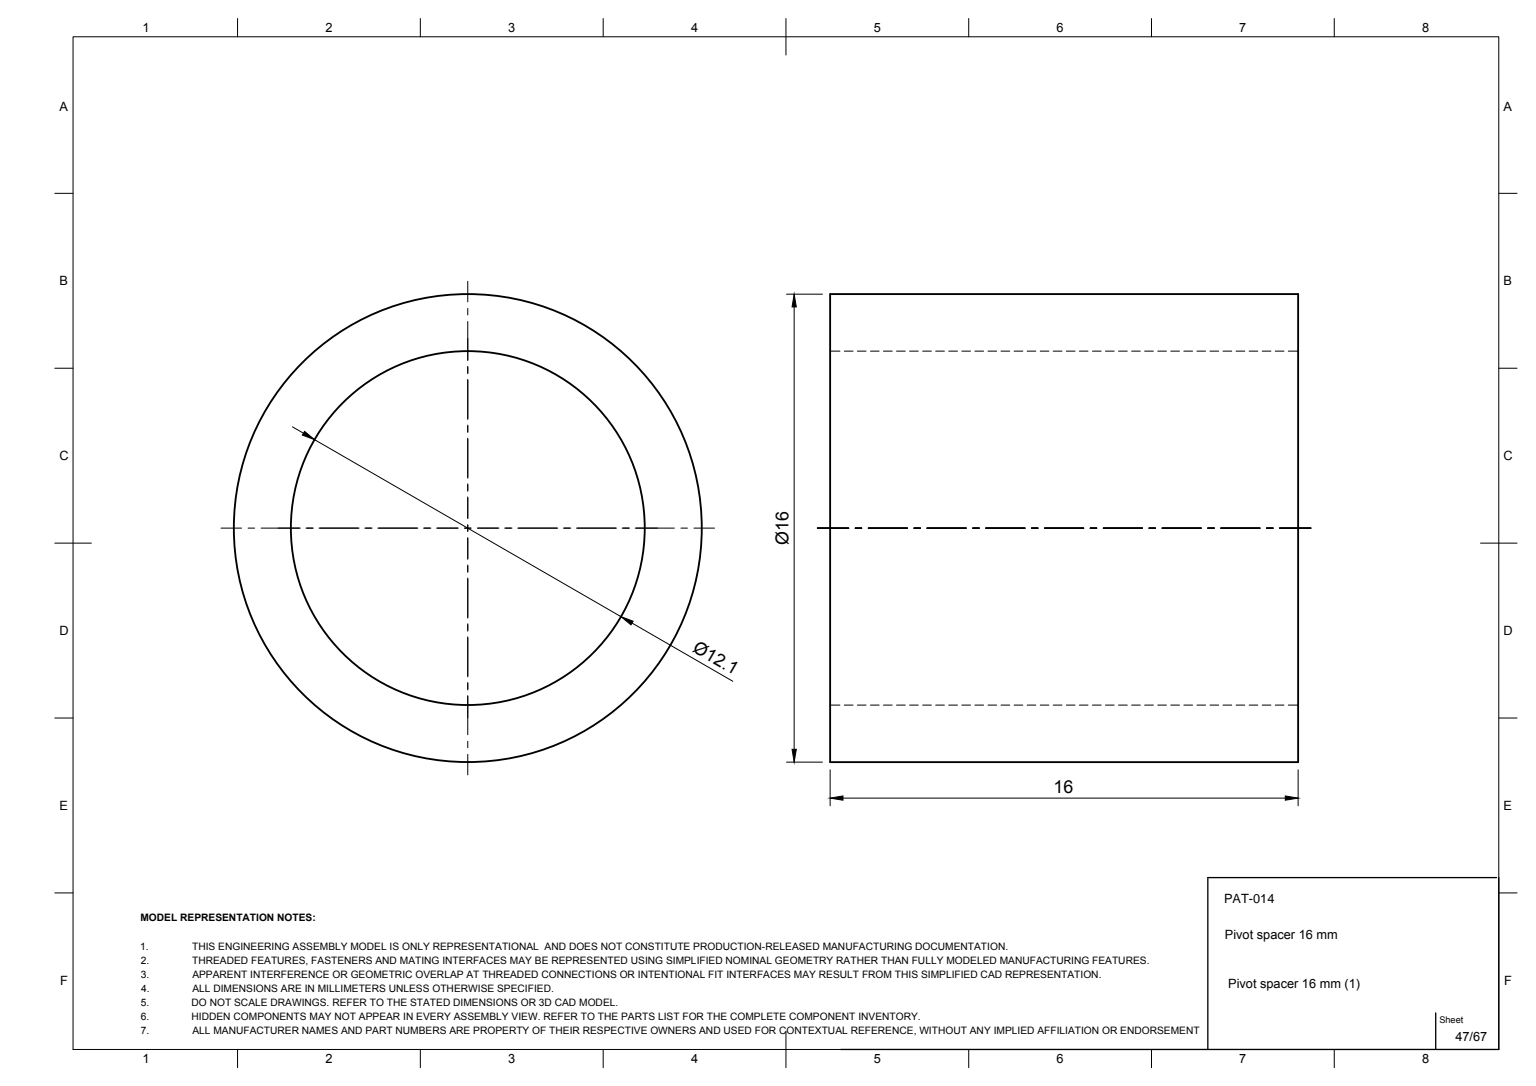
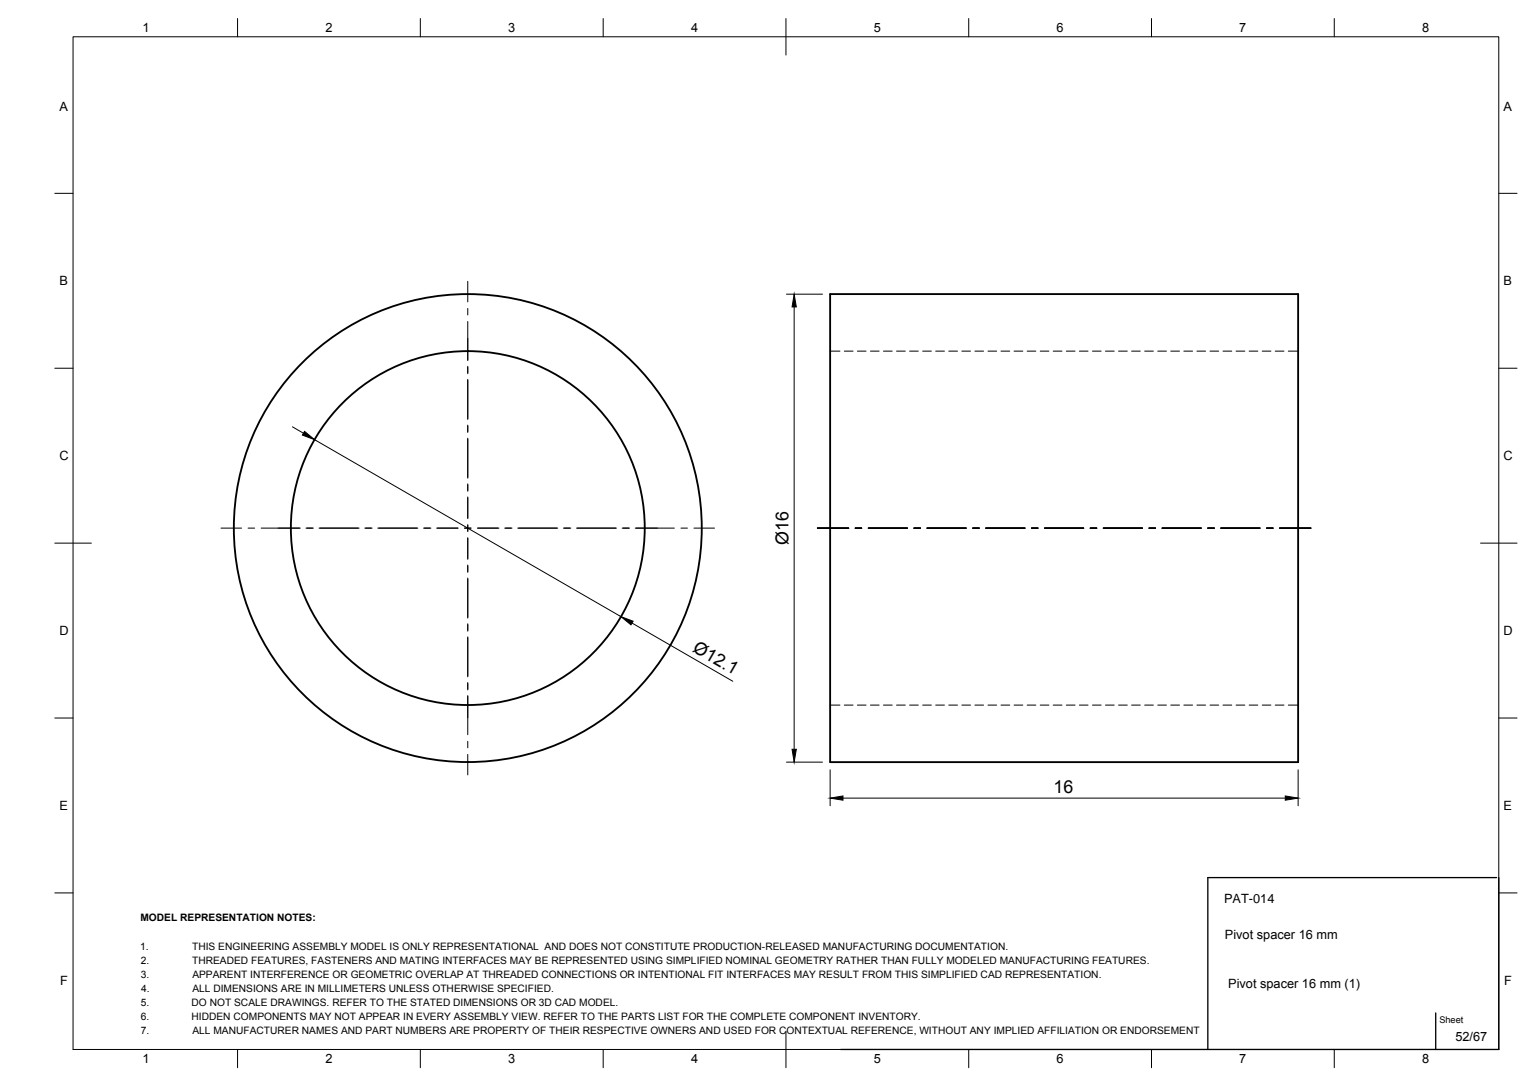
ISO-10303-21;
HEADER;
/* Generated by software containing ST-Developer
 * from STEP Tools, Inc. (www.steptools.com) 
 */

FILE_DESCRIPTION(
/* description */ ('Bin tilter linkage'),
/* implementation_level */ '2;1');

FILE_NAME(
/* name */ 'Pivot spacer 16 mm.step',
/* time_stamp */ '2026-10-28T03:26:24-07:00',
/* author */ (''),
/* organization */ (''),
/* preprocessor_version */ 'ST-DEVELOPER v20.2',
/* originating_system */ 'Autodesk Translation Framework v15.17.0.0',
/* authorisation */ '');

FILE_SCHEMA (('AUTOMOTIVE_DESIGN { 1 0 10303 214 3 1 1 }'));
ENDSEC;

DATA;
#10=MECHANICAL_DESIGN_GEOMETRIC_PRESENTATION_REPRESENTATION('',(#951),#23728);
#731=SHAPE_REPRESENTATION_RELATIONSHIP('SRR','None',#24199,#837);
#837=ADVANCED_BREP_SHAPE_REPRESENTATION('',(#1064),#23699);
#951=STYLED_ITEM('',(#24779),#1064);
#1064=MANIFOLD_SOLID_BREP('Body1',#12482);
#1420=FACE_BOUND('',#3607,.T.);
#1421=FACE_BOUND('',#3609,.T.);
#1786=PLANE('',#15046);
#1787=PLANE('',#15047);
#2494=FACE_OUTER_BOUND('',#3604,.T.);
#2495=FACE_OUTER_BOUND('',#3605,.T.);
#2496=FACE_OUTER_BOUND('',#3606,.T.);
#2497=FACE_OUTER_BOUND('',#3608,.T.);
#3604=EDGE_LOOP('',(#10639,#10640,#10641,#10642));
#3605=EDGE_LOOP('',(#10643,#10644,#10645,#10646));
#3606=EDGE_LOOP('',(#10647));
#3607=EDGE_LOOP('',(#10648));
#3608=EDGE_LOOP('',(#10649));
#3609=EDGE_LOOP('',(#10650));
#4347=LINE('',#22681,#5022);
#4348=LINE('',#22687,#5023);
#5022=VECTOR('',#18704,0.605);
#5023=VECTOR('',#18711,0.800000000000001);
#5820=CIRCLE('',#15041,0.605);
#5821=CIRCLE('',#15042,0.605);
#5822=CIRCLE('',#15044,0.800000000000001);
#5823=CIRCLE('',#15045,0.800000000000001);
#6719=VERTEX_POINT('',#22678);
#6720=VERTEX_POINT('',#22680);
#6721=VERTEX_POINT('',#22684);
#6722=VERTEX_POINT('',#22686);
#8059=EDGE_CURVE('',#6719,#6719,#5820,.T.);
#8060=EDGE_CURVE('',#6719,#6720,#4347,.T.);
#8061=EDGE_CURVE('',#6720,#6720,#5821,.T.);
#8062=EDGE_CURVE('',#6721,#6721,#5822,.T.);
#8063=EDGE_CURVE('',#6721,#6722,#4348,.T.);
#8064=EDGE_CURVE('',#6722,#6722,#5823,.T.);
#10639=ORIENTED_EDGE('',*,*,#8059,.F.);
#10640=ORIENTED_EDGE('',*,*,#8060,.T.);
#10641=ORIENTED_EDGE('',*,*,#8061,.T.);
#10642=ORIENTED_EDGE('',*,*,#8060,.F.);
#10643=ORIENTED_EDGE('',*,*,#8062,.F.);
#10644=ORIENTED_EDGE('',*,*,#8063,.T.);
#10645=ORIENTED_EDGE('',*,*,#8064,.T.);
#10646=ORIENTED_EDGE('',*,*,#8063,.F.);
#10647=ORIENTED_EDGE('',*,*,#8062,.T.);
#10648=ORIENTED_EDGE('',*,*,#8059,.T.);
#10649=ORIENTED_EDGE('',*,*,#8064,.F.);
#10650=ORIENTED_EDGE('',*,*,#8061,.F.);
#11553=CYLINDRICAL_SURFACE('',#15040,0.605);
#11554=CYLINDRICAL_SURFACE('',#15043,0.800000000000001);
#12219=ADVANCED_FACE('',(#2494),#11553,.F.);
#12220=ADVANCED_FACE('',(#2495),#11554,.T.);
#12221=ADVANCED_FACE('',(#2496,#1420),#1786,.T.);
#12222=ADVANCED_FACE('',(#2497,#1421),#1787,.F.);
#12482=CLOSED_SHELL('',(#12219,#12220,#12221,#12222));
#15039=AXIS2_PLACEMENT_3D('',#22676,#18698,#18699);
#15040=AXIS2_PLACEMENT_3D('',#22677,#18700,#18701);
#15041=AXIS2_PLACEMENT_3D('',#22679,#18702,#18703);
#15042=AXIS2_PLACEMENT_3D('',#22682,#18705,#18706);
#15043=AXIS2_PLACEMENT_3D('',#22683,#18707,#18708);
#15044=AXIS2_PLACEMENT_3D('',#22685,#18709,#18710);
#15045=AXIS2_PLACEMENT_3D('',#22688,#18712,#18713);
#15046=AXIS2_PLACEMENT_3D('',#22689,#18714,#18715);
#15047=AXIS2_PLACEMENT_3D('',#22690,#18716,#18717);
#18698=DIRECTION('axis',(0.,0.,1.));
#18699=DIRECTION('refdir',(1.,0.,0.));
#18700=DIRECTION('center_axis',(0.,1.,0.));
#18701=DIRECTION('ref_axis',(1.,0.,0.));
#18702=DIRECTION('center_axis',(0.,-1.,0.));
#18703=DIRECTION('ref_axis',(1.,0.,0.));
#18704=DIRECTION('',(0.,-1.,0.));
#18705=DIRECTION('center_axis',(0.,-1.,0.));
#18706=DIRECTION('ref_axis',(1.,0.,0.));
#18707=DIRECTION('center_axis',(0.,1.,0.));
#18708=DIRECTION('ref_axis',(1.,0.,0.));
#18709=DIRECTION('center_axis',(0.,1.,0.));
#18710=DIRECTION('ref_axis',(1.,0.,0.));
#18711=DIRECTION('',(0.,-1.,0.));
#18712=DIRECTION('center_axis',(0.,1.,0.));
#18713=DIRECTION('ref_axis',(1.,0.,0.));
#18714=DIRECTION('center_axis',(0.,1.,0.));
#18715=DIRECTION('ref_axis',(1.,0.,0.));
#18716=DIRECTION('center_axis',(0.,1.,0.));
#18717=DIRECTION('ref_axis',(1.,0.,0.));
#22676=CARTESIAN_POINT('',(0.,0.,0.));
#22677=CARTESIAN_POINT('Origin',(9.39692620785909,0.5,18.4202014332567));
#22678=CARTESIAN_POINT('',(8.79192620785908,2.1,18.4202014332567));
#22679=CARTESIAN_POINT('Origin',(9.39692620785909,2.1,18.4202014332567));
#22680=CARTESIAN_POINT('',(8.79192620785908,0.5,18.4202014332567));
#22681=CARTESIAN_POINT('',(8.79192620785908,0.5,18.4202014332567));
#22682=CARTESIAN_POINT('Origin',(9.39692620785909,0.5,18.4202014332567));
#22683=CARTESIAN_POINT('Origin',(9.39692620785909,0.5,18.4202014332567));
#22684=CARTESIAN_POINT('',(8.59692620785908,2.1,18.4202014332567));
#22685=CARTESIAN_POINT('Origin',(9.39692620785909,2.1,18.4202014332567));
#22686=CARTESIAN_POINT('',(8.59692620785908,0.5,18.4202014332567));
#22687=CARTESIAN_POINT('',(8.59692620785908,0.5,18.4202014332567));
#22688=CARTESIAN_POINT('Origin',(9.39692620785909,0.5,18.4202014332567));
#22689=CARTESIAN_POINT('Origin',(9.39692620785909,2.1,18.4202014332567));
#22690=CARTESIAN_POINT('Origin',(9.39692620785909,0.5,18.4202014332567));
#23582=UNCERTAINTY_MEASURE_WITH_UNIT(LENGTH_MEASURE(0.001),#23729,
'DISTANCE_ACCURACY_VALUE',
'Maximum model space distance between geometric entities at asserted c
onnectivities');
#23611=UNCERTAINTY_MEASURE_WITH_UNIT(LENGTH_MEASURE(0.001),#23729,
'DISTANCE_ACCURACY_VALUE',
'Maximum model space distance between geometric entities at asserted c
onnectivities');
#23699=(
GEOMETRIC_REPRESENTATION_CONTEXT(3)
GLOBAL_UNCERTAINTY_ASSIGNED_CONTEXT((#23582))
GLOBAL_UNIT_ASSIGNED_CONTEXT((#23729,#23731,#23732))
REPRESENTATION_CONTEXT('','3D')
);
#23728=(
GEOMETRIC_REPRESENTATION_CONTEXT(3)
GLOBAL_UNCERTAINTY_ASSIGNED_CONTEXT((#23611))
GLOBAL_UNIT_ASSIGNED_CONTEXT((#23729,#23731,#23732))
REPRESENTATION_CONTEXT('','3D')
);
#23729=(
LENGTH_UNIT()
NAMED_UNIT(*)
SI_UNIT(.CENTI.,.METRE.)
);
#23731=(
NAMED_UNIT(*)
PLANE_ANGLE_UNIT()
SI_UNIT($,.RADIAN.)
);
#23732=(
NAMED_UNIT(*)
SI_UNIT($,.STERADIAN.)
SOLID_ANGLE_UNIT()
);
#23820=SHAPE_DEFINITION_REPRESENTATION(#23987,#24199);
#23987=PRODUCT_DEFINITION_SHAPE('',$,#24316);
#24199=SHAPE_REPRESENTATION('',(#15039),#23699);
#24228=PRODUCT_DEFINITION_CONTEXT('part definition',#24578,'design');
#24316=PRODUCT_DEFINITION('Pivot spacer 16 mm','Pivot spacer 16 mm',#24432,
#24228);
#24432=PRODUCT_DEFINITION_FORMATION('',$,#24667);
#24578=APPLICATION_CONTEXT(
'Core Data for Automotive Mechanical Design Process');
#24579=PRODUCT_CONTEXT('part definition',#24578,'mechanical');
#24667=PRODUCT('Pivot spacer 16 mm','Pivot spacer 16 mm',
'Pivot spacer 16 mm',(#24579));
#24773=COLOUR_RGB('Off White',0.89,0.88,0.83);
#24774=FILL_AREA_STYLE_COLOUR('',#24773);
#24775=FILL_AREA_STYLE('',(#24774));
#24776=SURFACE_STYLE_FILL_AREA(#24775);
#24777=SURFACE_SIDE_STYLE('',(#24776));
#24778=SURFACE_STYLE_USAGE(.BOTH.,#24777);
#24779=PRESENTATION_STYLE_ASSIGNMENT((#24778));
ENDSEC;
END-ISO-10303-21;
